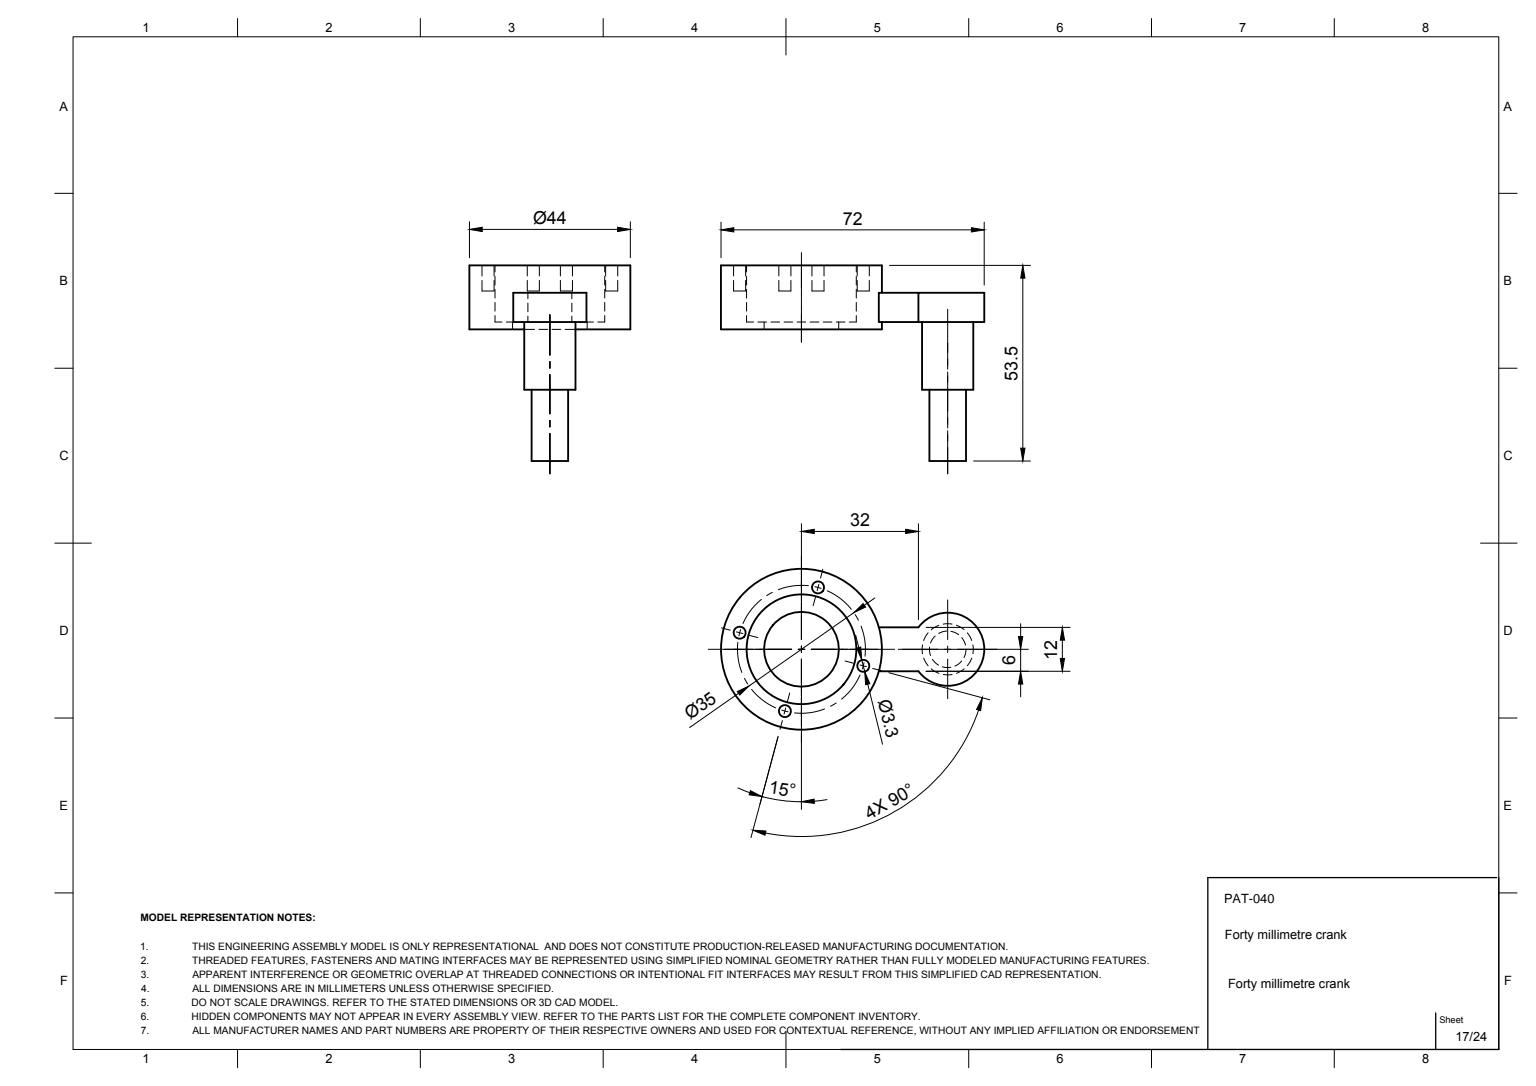
ISO-10303-21;
HEADER;
/* Generated by software containing ST-Developer
 * from STEP Tools, Inc. (www.steptools.com) 
 */

FILE_DESCRIPTION(
/* description */ ('Four-bar tabletop demonstrator'),
/* implementation_level */ '2;1');

FILE_NAME(
/* name */ 'Forty millimetre crank.step',
/* time_stamp */ '2026-10-29T17:05:23-07:00',
/* author */ (''),
/* organization */ (''),
/* preprocessor_version */ 'ST-DEVELOPER v20.2',
/* originating_system */ 'Autodesk Translation Framework v15.17.0.0',
/* authorisation */ '');

FILE_SCHEMA (('AUTOMOTIVE_DESIGN { 1 0 10303 214 3 1 1 }'));
ENDSEC;

DATA;
#10=MECHANICAL_DESIGN_GEOMETRIC_PRESENTATION_REPRESENTATION('',(#340),#6705);
#310=SHAPE_REPRESENTATION_RELATIONSHIP('SRR','None',#6818,#325);
#325=ADVANCED_BREP_SHAPE_REPRESENTATION('',(#362),#6691);
#340=STYLED_ITEM('',(#7003),#362);
#362=MANIFOLD_SOLID_BREP('Body1',#3385);
#416=FACE_BOUND('',#869,.T.);
#417=FACE_BOUND('',#872,.T.);
#418=FACE_BOUND('',#874,.T.);
#419=FACE_BOUND('',#875,.T.);
#420=FACE_BOUND('',#876,.T.);
#421=FACE_BOUND('',#877,.T.);
#422=FACE_BOUND('',#878,.T.);
#423=FACE_BOUND('',#880,.T.);
#424=FACE_BOUND('',#886,.T.);
#425=FACE_BOUND('',#888,.T.);
#491=PLANE('',#3705);
#492=PLANE('',#3709);
#493=PLANE('',#3713);
#494=PLANE('',#3717);
#495=PLANE('',#3721);
#496=PLANE('',#3730);
#497=PLANE('',#3731);
#498=PLANE('',#3732);
#499=PLANE('',#3733);
#500=PLANE('',#3735);
#501=PLANE('',#3738);
#502=PLANE('',#3740);
#503=PLANE('',#3746);
#621=FACE_OUTER_BOUND('',#859,.T.);
#622=FACE_OUTER_BOUND('',#860,.T.);
#623=FACE_OUTER_BOUND('',#861,.T.);
#624=FACE_OUTER_BOUND('',#862,.T.);
#625=FACE_OUTER_BOUND('',#863,.T.);
#626=FACE_OUTER_BOUND('',#864,.T.);
#627=FACE_OUTER_BOUND('',#865,.T.);
#628=FACE_OUTER_BOUND('',#866,.T.);
#629=FACE_OUTER_BOUND('',#867,.T.);
#630=FACE_OUTER_BOUND('',#868,.T.);
#631=FACE_OUTER_BOUND('',#870,.T.);
#632=FACE_OUTER_BOUND('',#871,.T.);
#633=FACE_OUTER_BOUND('',#873,.T.);
#634=FACE_OUTER_BOUND('',#879,.T.);
#635=FACE_OUTER_BOUND('',#881,.T.);
#636=FACE_OUTER_BOUND('',#882,.T.);
#637=FACE_OUTER_BOUND('',#883,.T.);
#638=FACE_OUTER_BOUND('',#884,.T.);
#639=FACE_OUTER_BOUND('',#885,.T.);
#640=FACE_OUTER_BOUND('',#887,.T.);
#641=FACE_OUTER_BOUND('',#889,.T.);
#642=FACE_OUTER_BOUND('',#890,.T.);
#643=FACE_OUTER_BOUND('',#891,.T.);
#859=EDGE_LOOP('',(#2550,#2551,#2552,#2553));
#860=EDGE_LOOP('',(#2554));
#861=EDGE_LOOP('',(#2555,#2556,#2557,#2558));
#862=EDGE_LOOP('',(#2559));
#863=EDGE_LOOP('',(#2560,#2561,#2562,#2563));
#864=EDGE_LOOP('',(#2564));
#865=EDGE_LOOP('',(#2565,#2566,#2567,#2568));
#866=EDGE_LOOP('',(#2569));
#867=EDGE_LOOP('',(#2570,#2571,#2572,#2573));
#868=EDGE_LOOP('',(#2574));
#869=EDGE_LOOP('',(#2575));
#870=EDGE_LOOP('',(#2576,#2577,#2578,#2579));
#871=EDGE_LOOP('',(#2580,#2581,#2582,#2583));
#872=EDGE_LOOP('',(#2584,#2585,#2586,#2587));
#873=EDGE_LOOP('',(#2588));
#874=EDGE_LOOP('',(#2589));
#875=EDGE_LOOP('',(#2590));
#876=EDGE_LOOP('',(#2591));
#877=EDGE_LOOP('',(#2592));
#878=EDGE_LOOP('',(#2593));
#879=EDGE_LOOP('',(#2594));
#880=EDGE_LOOP('',(#2595));
#881=EDGE_LOOP('',(#2596,#2597,#2598,#2599));
#882=EDGE_LOOP('',(#2600,#2601,#2602,#2603));
#883=EDGE_LOOP('',(#2604,#2605,#2606,#2607));
#884=EDGE_LOOP('',(#2608,#2609,#2610,#2611));
#885=EDGE_LOOP('',(#2612,#2613,#2614,#2615));
#886=EDGE_LOOP('',(#2616));
#887=EDGE_LOOP('',(#2617));
#888=EDGE_LOOP('',(#2618));
#889=EDGE_LOOP('',(#2619,#2620,#2621,#2622));
#890=EDGE_LOOP('',(#2623,#2624,#2625,#2626));
#891=EDGE_LOOP('',(#2627));
#1113=LINE('',#5581,#1283);
#1114=LINE('',#5588,#1284);
#1115=LINE('',#5595,#1285);
#1116=LINE('',#5602,#1286);
#1117=LINE('',#5609,#1287);
#1118=LINE('',#5617,#1288);
#1119=LINE('',#5622,#1289);
#1120=LINE('',#5626,#1290);
#1121=LINE('',#5630,#1291);
#1122=LINE('',#5636,#1292);
#1123=LINE('',#5638,#1293);
#1124=LINE('',#5639,#1294);
#1125=LINE('',#5642,#1295);
#1126=LINE('',#5646,#1296);
#1127=LINE('',#5647,#1297);
#1128=LINE('',#5659,#1298);
#1129=LINE('',#5662,#1299);
#1283=VECTOR('',#4394,0.165);
#1284=VECTOR('',#4403,0.165);
#1285=VECTOR('',#4412,0.165);
#1286=VECTOR('',#4421,0.165);
#1287=VECTOR('',#4430,1.5);
#1288=VECTOR('',#4441,1.02);
#1289=VECTOR('',#4446,2.2);
#1290=VECTOR('',#4449,1.);
#1291=VECTOR('',#4452,1.);
#1292=VECTOR('',#4461,1.);
#1293=VECTOR('',#4462,1.);
#1294=VECTOR('',#4463,1.);
#1295=VECTOR('',#4466,1.);
#1296=VECTOR('',#4471,1.);
#1297=VECTOR('',#4472,1.);
#1298=VECTOR('',#4489,0.7);
#1299=VECTOR('',#4492,0.5);
#1452=CIRCLE('',#3703,0.165);
#1453=CIRCLE('',#3704,0.165);
#1454=CIRCLE('',#3707,0.165);
#1455=CIRCLE('',#3708,0.165);
#1456=CIRCLE('',#3711,0.165);
#1457=CIRCLE('',#3712,0.165);
#1458=CIRCLE('',#3715,0.165);
#1459=CIRCLE('',#3716,0.165);
#1460=CIRCLE('',#3719,1.5);
#1461=CIRCLE('',#3720,1.5);
#1462=CIRCLE('',#3722,1.02);
#1463=CIRCLE('',#3724,1.02);
#1464=CIRCLE('',#3726,2.2);
#1465=CIRCLE('',#3727,2.2);
#1466=CIRCLE('',#3728,2.2);
#1467=CIRCLE('',#3729,2.2);
#1468=CIRCLE('',#3734,1.);
#1469=CIRCLE('',#3737,1.);
#1470=CIRCLE('',#3739,0.7);
#1471=CIRCLE('',#3741,0.7);
#1472=CIRCLE('',#3742,0.5);
#1473=CIRCLE('',#3745,0.5);
#1687=VERTEX_POINT('',#5578);
#1688=VERTEX_POINT('',#5580);
#1689=VERTEX_POINT('',#5585);
#1690=VERTEX_POINT('',#5587);
#1691=VERTEX_POINT('',#5592);
#1692=VERTEX_POINT('',#5594);
#1693=VERTEX_POINT('',#5599);
#1694=VERTEX_POINT('',#5601);
#1695=VERTEX_POINT('',#5606);
#1696=VERTEX_POINT('',#5608);
#1697=VERTEX_POINT('',#5612);
#1698=VERTEX_POINT('',#5615);
#1699=VERTEX_POINT('',#5619);
#1700=VERTEX_POINT('',#5621);
#1701=VERTEX_POINT('',#5624);
#1702=VERTEX_POINT('',#5625);
#1703=VERTEX_POINT('',#5627);
#1704=VERTEX_POINT('',#5629);
#1705=VERTEX_POINT('',#5635);
#1706=VERTEX_POINT('',#5637);
#1707=VERTEX_POINT('',#5641);
#1708=VERTEX_POINT('',#5645);
#1709=VERTEX_POINT('',#5651);
#1710=VERTEX_POINT('',#5654);
#1711=VERTEX_POINT('',#5656);
#1712=VERTEX_POINT('',#5661);
#2011=EDGE_CURVE('',#1687,#1687,#1452,.T.);
#2012=EDGE_CURVE('',#1687,#1688,#1113,.T.);
#2013=EDGE_CURVE('',#1688,#1688,#1453,.T.);
#2014=EDGE_CURVE('',#1689,#1689,#1454,.T.);
#2015=EDGE_CURVE('',#1689,#1690,#1114,.T.);
#2016=EDGE_CURVE('',#1690,#1690,#1455,.T.);
#2017=EDGE_CURVE('',#1691,#1691,#1456,.T.);
#2018=EDGE_CURVE('',#1691,#1692,#1115,.T.);
#2019=EDGE_CURVE('',#1692,#1692,#1457,.T.);
#2020=EDGE_CURVE('',#1693,#1693,#1458,.T.);
#2021=EDGE_CURVE('',#1693,#1694,#1116,.T.);
#2022=EDGE_CURVE('',#1694,#1694,#1459,.T.);
#2023=EDGE_CURVE('',#1695,#1695,#1460,.T.);
#2024=EDGE_CURVE('',#1695,#1696,#1117,.T.);
#2025=EDGE_CURVE('',#1696,#1696,#1461,.T.);
#2026=EDGE_CURVE('',#1697,#1697,#1462,.T.);
#2027=EDGE_CURVE('',#1698,#1698,#1463,.T.);
#2028=EDGE_CURVE('',#1698,#1697,#1118,.T.);
#2029=EDGE_CURVE('',#1699,#1699,#1464,.T.);
#2030=EDGE_CURVE('',#1699,#1700,#1119,.T.);
#2031=EDGE_CURVE('',#1700,#1700,#1465,.T.);
#2032=EDGE_CURVE('',#1701,#1702,#1120,.T.);
#2033=EDGE_CURVE('',#1703,#1701,#1466,.T.);
#2034=EDGE_CURVE('',#1704,#1703,#1121,.T.);
#2035=EDGE_CURVE('',#1702,#1704,#1467,.T.);
#2036=EDGE_CURVE('',#1705,#1703,#1122,.T.);
#2037=EDGE_CURVE('',#1706,#1705,#1123,.T.);
#2038=EDGE_CURVE('',#1704,#1706,#1124,.T.);
#2039=EDGE_CURVE('',#1701,#1707,#1125,.T.);
#2040=EDGE_CURVE('',#1707,#1705,#1468,.T.);
#2041=EDGE_CURVE('',#1708,#1702,#1126,.T.);
#2042=EDGE_CURVE('',#1707,#1708,#1127,.T.);
#2043=EDGE_CURVE('',#1708,#1706,#1469,.T.);
#2044=EDGE_CURVE('',#1709,#1709,#1470,.T.);
#2045=EDGE_CURVE('',#1710,#1710,#1471,.T.);
#2046=EDGE_CURVE('',#1711,#1711,#1472,.T.);
#2047=EDGE_CURVE('',#1709,#1710,#1128,.T.);
#2048=EDGE_CURVE('',#1711,#1712,#1129,.T.);
#2049=EDGE_CURVE('',#1712,#1712,#1473,.T.);
#2550=ORIENTED_EDGE('',*,*,#2011,.F.);
#2551=ORIENTED_EDGE('',*,*,#2012,.T.);
#2552=ORIENTED_EDGE('',*,*,#2013,.F.);
#2553=ORIENTED_EDGE('',*,*,#2012,.F.);
#2554=ORIENTED_EDGE('',*,*,#2011,.T.);
#2555=ORIENTED_EDGE('',*,*,#2014,.F.);
#2556=ORIENTED_EDGE('',*,*,#2015,.T.);
#2557=ORIENTED_EDGE('',*,*,#2016,.F.);
#2558=ORIENTED_EDGE('',*,*,#2015,.F.);
#2559=ORIENTED_EDGE('',*,*,#2014,.T.);
#2560=ORIENTED_EDGE('',*,*,#2017,.F.);
#2561=ORIENTED_EDGE('',*,*,#2018,.T.);
#2562=ORIENTED_EDGE('',*,*,#2019,.F.);
#2563=ORIENTED_EDGE('',*,*,#2018,.F.);
#2564=ORIENTED_EDGE('',*,*,#2017,.T.);
#2565=ORIENTED_EDGE('',*,*,#2020,.F.);
#2566=ORIENTED_EDGE('',*,*,#2021,.T.);
#2567=ORIENTED_EDGE('',*,*,#2022,.F.);
#2568=ORIENTED_EDGE('',*,*,#2021,.F.);
#2569=ORIENTED_EDGE('',*,*,#2020,.T.);
#2570=ORIENTED_EDGE('',*,*,#2023,.F.);
#2571=ORIENTED_EDGE('',*,*,#2024,.T.);
#2572=ORIENTED_EDGE('',*,*,#2025,.F.);
#2573=ORIENTED_EDGE('',*,*,#2024,.F.);
#2574=ORIENTED_EDGE('',*,*,#2023,.T.);
#2575=ORIENTED_EDGE('',*,*,#2026,.F.);
#2576=ORIENTED_EDGE('',*,*,#2027,.F.);
#2577=ORIENTED_EDGE('',*,*,#2028,.T.);
#2578=ORIENTED_EDGE('',*,*,#2026,.T.);
#2579=ORIENTED_EDGE('',*,*,#2028,.F.);
#2580=ORIENTED_EDGE('',*,*,#2029,.F.);
#2581=ORIENTED_EDGE('',*,*,#2030,.T.);
#2582=ORIENTED_EDGE('',*,*,#2031,.T.);
#2583=ORIENTED_EDGE('',*,*,#2030,.F.);
#2584=ORIENTED_EDGE('',*,*,#2032,.F.);
#2585=ORIENTED_EDGE('',*,*,#2033,.F.);
#2586=ORIENTED_EDGE('',*,*,#2034,.F.);
#2587=ORIENTED_EDGE('',*,*,#2035,.F.);
#2588=ORIENTED_EDGE('',*,*,#2029,.T.);
#2589=ORIENTED_EDGE('',*,*,#2025,.T.);
#2590=ORIENTED_EDGE('',*,*,#2022,.T.);
#2591=ORIENTED_EDGE('',*,*,#2019,.T.);
#2592=ORIENTED_EDGE('',*,*,#2016,.T.);
#2593=ORIENTED_EDGE('',*,*,#2013,.T.);
#2594=ORIENTED_EDGE('',*,*,#2031,.F.);
#2595=ORIENTED_EDGE('',*,*,#2027,.T.);
#2596=ORIENTED_EDGE('',*,*,#2034,.T.);
#2597=ORIENTED_EDGE('',*,*,#2036,.F.);
#2598=ORIENTED_EDGE('',*,*,#2037,.F.);
#2599=ORIENTED_EDGE('',*,*,#2038,.F.);
#2600=ORIENTED_EDGE('',*,*,#2033,.T.);
#2601=ORIENTED_EDGE('',*,*,#2039,.T.);
#2602=ORIENTED_EDGE('',*,*,#2040,.T.);
#2603=ORIENTED_EDGE('',*,*,#2036,.T.);
#2604=ORIENTED_EDGE('',*,*,#2032,.T.);
#2605=ORIENTED_EDGE('',*,*,#2041,.F.);
#2606=ORIENTED_EDGE('',*,*,#2042,.F.);
#2607=ORIENTED_EDGE('',*,*,#2039,.F.);
#2608=ORIENTED_EDGE('',*,*,#2042,.T.);
#2609=ORIENTED_EDGE('',*,*,#2043,.T.);
#2610=ORIENTED_EDGE('',*,*,#2037,.T.);
#2611=ORIENTED_EDGE('',*,*,#2040,.F.);
#2612=ORIENTED_EDGE('',*,*,#2035,.T.);
#2613=ORIENTED_EDGE('',*,*,#2038,.T.);
#2614=ORIENTED_EDGE('',*,*,#2043,.F.);
#2615=ORIENTED_EDGE('',*,*,#2041,.T.);
#2616=ORIENTED_EDGE('',*,*,#2044,.T.);
#2617=ORIENTED_EDGE('',*,*,#2045,.F.);
#2618=ORIENTED_EDGE('',*,*,#2046,.F.);
#2619=ORIENTED_EDGE('',*,*,#2044,.F.);
#2620=ORIENTED_EDGE('',*,*,#2047,.T.);
#2621=ORIENTED_EDGE('',*,*,#2045,.T.);
#2622=ORIENTED_EDGE('',*,*,#2047,.F.);
#2623=ORIENTED_EDGE('',*,*,#2046,.T.);
#2624=ORIENTED_EDGE('',*,*,#2048,.T.);
#2625=ORIENTED_EDGE('',*,*,#2049,.T.);
#2626=ORIENTED_EDGE('',*,*,#2048,.F.);
#2627=ORIENTED_EDGE('',*,*,#2049,.F.);
#3131=CYLINDRICAL_SURFACE('',#3702,0.165);
#3132=CYLINDRICAL_SURFACE('',#3706,0.165);
#3133=CYLINDRICAL_SURFACE('',#3710,0.165);
#3134=CYLINDRICAL_SURFACE('',#3714,0.165);
#3135=CYLINDRICAL_SURFACE('',#3718,1.5);
#3136=CYLINDRICAL_SURFACE('',#3723,1.02);
#3137=CYLINDRICAL_SURFACE('',#3725,2.2);
#3138=CYLINDRICAL_SURFACE('',#3736,1.);
#3139=CYLINDRICAL_SURFACE('',#3743,0.7);
#3140=CYLINDRICAL_SURFACE('',#3744,0.5);
#3237=ADVANCED_FACE('',(#621),#3131,.F.);
#3238=ADVANCED_FACE('',(#622),#491,.T.);
#3239=ADVANCED_FACE('',(#623),#3132,.F.);
#3240=ADVANCED_FACE('',(#624),#492,.T.);
#3241=ADVANCED_FACE('',(#625),#3133,.F.);
#3242=ADVANCED_FACE('',(#626),#493,.T.);
#3243=ADVANCED_FACE('',(#627),#3134,.F.);
#3244=ADVANCED_FACE('',(#628),#494,.T.);
#3245=ADVANCED_FACE('',(#629),#3135,.F.);
#3246=ADVANCED_FACE('',(#630,#416),#495,.T.);
#3247=ADVANCED_FACE('',(#631),#3136,.F.);
#3248=ADVANCED_FACE('',(#632,#417),#3137,.T.);
#3249=ADVANCED_FACE('',(#633,#418,#419,#420,#421,#422),#496,.T.);
#3250=ADVANCED_FACE('',(#634,#423),#497,.F.);
#3251=ADVANCED_FACE('',(#635),#498,.T.);
#3252=ADVANCED_FACE('',(#636),#499,.T.);
#3253=ADVANCED_FACE('',(#637),#500,.T.);
#3254=ADVANCED_FACE('',(#638),#3138,.T.);
#3255=ADVANCED_FACE('',(#639,#424),#501,.F.);
#3256=ADVANCED_FACE('',(#640,#425),#502,.F.);
#3257=ADVANCED_FACE('',(#641),#3139,.T.);
#3258=ADVANCED_FACE('',(#642),#3140,.T.);
#3259=ADVANCED_FACE('',(#643),#503,.F.);
#3385=CLOSED_SHELL('',(#3237,#3238,#3239,#3240,#3241,#3242,#3243,#3244,
#3245,#3246,#3247,#3248,#3249,#3250,#3251,#3252,#3253,#3254,#3255,#3256,
#3257,#3258,#3259));
#3701=AXIS2_PLACEMENT_3D('',#5576,#4388,#4389);
#3702=AXIS2_PLACEMENT_3D('',#5577,#4390,#4391);
#3703=AXIS2_PLACEMENT_3D('',#5579,#4392,#4393);
#3704=AXIS2_PLACEMENT_3D('',#5582,#4395,#4396);
#3705=AXIS2_PLACEMENT_3D('',#5583,#4397,#4398);
#3706=AXIS2_PLACEMENT_3D('',#5584,#4399,#4400);
#3707=AXIS2_PLACEMENT_3D('',#5586,#4401,#4402);
#3708=AXIS2_PLACEMENT_3D('',#5589,#4404,#4405);
#3709=AXIS2_PLACEMENT_3D('',#5590,#4406,#4407);
#3710=AXIS2_PLACEMENT_3D('',#5591,#4408,#4409);
#3711=AXIS2_PLACEMENT_3D('',#5593,#4410,#4411);
#3712=AXIS2_PLACEMENT_3D('',#5596,#4413,#4414);
#3713=AXIS2_PLACEMENT_3D('',#5597,#4415,#4416);
#3714=AXIS2_PLACEMENT_3D('',#5598,#4417,#4418);
#3715=AXIS2_PLACEMENT_3D('',#5600,#4419,#4420);
#3716=AXIS2_PLACEMENT_3D('',#5603,#4422,#4423);
#3717=AXIS2_PLACEMENT_3D('',#5604,#4424,#4425);
#3718=AXIS2_PLACEMENT_3D('',#5605,#4426,#4427);
#3719=AXIS2_PLACEMENT_3D('',#5607,#4428,#4429);
#3720=AXIS2_PLACEMENT_3D('',#5610,#4431,#4432);
#3721=AXIS2_PLACEMENT_3D('',#5611,#4433,#4434);
#3722=AXIS2_PLACEMENT_3D('',#5613,#4435,#4436);
#3723=AXIS2_PLACEMENT_3D('',#5614,#4437,#4438);
#3724=AXIS2_PLACEMENT_3D('',#5616,#4439,#4440);
#3725=AXIS2_PLACEMENT_3D('',#5618,#4442,#4443);
#3726=AXIS2_PLACEMENT_3D('',#5620,#4444,#4445);
#3727=AXIS2_PLACEMENT_3D('',#5623,#4447,#4448);
#3728=AXIS2_PLACEMENT_3D('',#5628,#4450,#4451);
#3729=AXIS2_PLACEMENT_3D('',#5631,#4453,#4454);
#3730=AXIS2_PLACEMENT_3D('',#5632,#4455,#4456);
#3731=AXIS2_PLACEMENT_3D('',#5633,#4457,#4458);
#3732=AXIS2_PLACEMENT_3D('',#5634,#4459,#4460);
#3733=AXIS2_PLACEMENT_3D('',#5640,#4464,#4465);
#3734=AXIS2_PLACEMENT_3D('',#5643,#4467,#4468);
#3735=AXIS2_PLACEMENT_3D('',#5644,#4469,#4470);
#3736=AXIS2_PLACEMENT_3D('',#5648,#4473,#4474);
#3737=AXIS2_PLACEMENT_3D('',#5649,#4475,#4476);
#3738=AXIS2_PLACEMENT_3D('',#5650,#4477,#4478);
#3739=AXIS2_PLACEMENT_3D('',#5652,#4479,#4480);
#3740=AXIS2_PLACEMENT_3D('',#5653,#4481,#4482);
#3741=AXIS2_PLACEMENT_3D('',#5655,#4483,#4484);
#3742=AXIS2_PLACEMENT_3D('',#5657,#4485,#4486);
#3743=AXIS2_PLACEMENT_3D('',#5658,#4487,#4488);
#3744=AXIS2_PLACEMENT_3D('',#5660,#4490,#4491);
#3745=AXIS2_PLACEMENT_3D('',#5663,#4493,#4494);
#3746=AXIS2_PLACEMENT_3D('',#5664,#4495,#4496);
#4388=DIRECTION('axis',(0.,0.,1.));
#4389=DIRECTION('refdir',(1.,0.,0.));
#4390=DIRECTION('center_axis',(0.,0.,1.));
#4391=DIRECTION('ref_axis',(1.,0.,0.));
#4392=DIRECTION('center_axis',(0.,0.,1.));
#4393=DIRECTION('ref_axis',(1.,0.,0.));
#4394=DIRECTION('',(0.,0.,1.));
#4395=DIRECTION('center_axis',(0.,0.,-1.));
#4396=DIRECTION('ref_axis',(1.,0.,0.));
#4397=DIRECTION('center_axis',(0.,0.,1.));
#4398=DIRECTION('ref_axis',(1.,0.,0.));
#4399=DIRECTION('center_axis',(0.,0.,1.));
#4400=DIRECTION('ref_axis',(1.,0.,0.));
#4401=DIRECTION('center_axis',(0.,0.,1.));
#4402=DIRECTION('ref_axis',(1.,0.,0.));
#4403=DIRECTION('',(0.,0.,1.));
#4404=DIRECTION('center_axis',(0.,0.,-1.));
#4405=DIRECTION('ref_axis',(1.,0.,0.));
#4406=DIRECTION('center_axis',(0.,0.,1.));
#4407=DIRECTION('ref_axis',(1.,0.,0.));
#4408=DIRECTION('center_axis',(0.,0.,1.));
#4409=DIRECTION('ref_axis',(1.,0.,0.));
#4410=DIRECTION('center_axis',(0.,0.,1.));
#4411=DIRECTION('ref_axis',(1.,0.,0.));
#4412=DIRECTION('',(0.,0.,1.));
#4413=DIRECTION('center_axis',(0.,0.,-1.));
#4414=DIRECTION('ref_axis',(1.,0.,0.));
#4415=DIRECTION('center_axis',(0.,0.,1.));
#4416=DIRECTION('ref_axis',(1.,0.,0.));
#4417=DIRECTION('center_axis',(0.,0.,1.));
#4418=DIRECTION('ref_axis',(1.,0.,0.));
#4419=DIRECTION('center_axis',(0.,0.,1.));
#4420=DIRECTION('ref_axis',(1.,0.,0.));
#4421=DIRECTION('',(0.,0.,1.));
#4422=DIRECTION('center_axis',(0.,0.,-1.));
#4423=DIRECTION('ref_axis',(1.,0.,0.));
#4424=DIRECTION('center_axis',(0.,0.,1.));
#4425=DIRECTION('ref_axis',(1.,0.,0.));
#4426=DIRECTION('center_axis',(0.,0.,1.));
#4427=DIRECTION('ref_axis',(1.,0.,0.));
#4428=DIRECTION('center_axis',(0.,0.,1.));
#4429=DIRECTION('ref_axis',(1.,0.,0.));
#4430=DIRECTION('',(0.,0.,1.));
#4431=DIRECTION('center_axis',(0.,0.,-1.));
#4432=DIRECTION('ref_axis',(1.,0.,0.));
#4433=DIRECTION('center_axis',(0.,0.,1.));
#4434=DIRECTION('ref_axis',(1.,0.,0.));
#4435=DIRECTION('center_axis',(0.,0.,1.));
#4436=DIRECTION('ref_axis',(1.,0.,0.));
#4437=DIRECTION('center_axis',(0.,0.,1.));
#4438=DIRECTION('ref_axis',(1.,0.,0.));
#4439=DIRECTION('center_axis',(0.,0.,1.));
#4440=DIRECTION('ref_axis',(1.,0.,0.));
#4441=DIRECTION('',(0.,0.,1.));
#4442=DIRECTION('center_axis',(0.,0.,1.));
#4443=DIRECTION('ref_axis',(1.,0.,0.));
#4444=DIRECTION('center_axis',(0.,0.,1.));
#4445=DIRECTION('ref_axis',(1.,0.,0.));
#4446=DIRECTION('',(0.,0.,-1.));
#4447=DIRECTION('center_axis',(0.,0.,1.));
#4448=DIRECTION('ref_axis',(1.,0.,0.));
#4449=DIRECTION('',(0.,0.,-1.));
#4450=DIRECTION('center_axis',(0.,0.,-1.));
#4451=DIRECTION('ref_axis',(1.,0.,0.));
#4452=DIRECTION('',(0.,0.,1.));
#4453=DIRECTION('center_axis',(0.,0.,1.));
#4454=DIRECTION('ref_axis',(1.,0.,0.));
#4455=DIRECTION('center_axis',(0.,0.,1.));
#4456=DIRECTION('ref_axis',(1.,0.,0.));
#4457=DIRECTION('center_axis',(0.,0.,1.));
#4458=DIRECTION('ref_axis',(1.,0.,0.));
#4459=DIRECTION('center_axis',(0.866025403784439,-0.5,0.));
#4460=DIRECTION('ref_axis',(0.5,0.866025403784439,0.));
#4461=DIRECTION('',(0.5,0.866025403784439,0.));
#4462=DIRECTION('',(0.,0.,1.));
#4463=DIRECTION('',(-0.5,-0.866025403784439,0.));
#4464=DIRECTION('center_axis',(0.,0.,1.));
#4465=DIRECTION('ref_axis',(1.,0.,0.));
#4466=DIRECTION('',(-0.5,-0.866025403784439,0.));
#4467=DIRECTION('center_axis',(0.,0.,1.));
#4468=DIRECTION('ref_axis',(1.,0.,0.));
#4469=DIRECTION('center_axis',(-0.866025403784439,0.5,0.));
#4470=DIRECTION('ref_axis',(-0.5,-0.866025403784439,0.));
#4471=DIRECTION('',(0.5,0.866025403784439,0.));
#4472=DIRECTION('',(0.,0.,-1.));
#4473=DIRECTION('center_axis',(0.,0.,1.));
#4474=DIRECTION('ref_axis',(-0.5,-0.866025403784438,0.));
#4475=DIRECTION('center_axis',(0.,0.,1.));
#4476=DIRECTION('ref_axis',(1.,0.,0.));
#4477=DIRECTION('center_axis',(0.,0.,1.));
#4478=DIRECTION('ref_axis',(1.,0.,0.));
#4479=DIRECTION('center_axis',(0.,0.,1.));
#4480=DIRECTION('ref_axis',(1.,0.,0.));
#4481=DIRECTION('center_axis',(0.,0.,1.));
#4482=DIRECTION('ref_axis',(1.,0.,0.));
#4483=DIRECTION('center_axis',(0.,0.,1.));
#4484=DIRECTION('ref_axis',(1.,0.,0.));
#4485=DIRECTION('center_axis',(0.,0.,-1.));
#4486=DIRECTION('ref_axis',(1.,0.,0.));
#4487=DIRECTION('center_axis',(0.,0.,1.));
#4488=DIRECTION('ref_axis',(1.,0.,0.));
#4489=DIRECTION('',(0.,0.,-1.));
#4490=DIRECTION('center_axis',(0.,0.,1.));
#4491=DIRECTION('ref_axis',(1.,0.,0.));
#4492=DIRECTION('',(0.,0.,-1.));
#4493=DIRECTION('center_axis',(0.,0.,1.));
#4494=DIRECTION('ref_axis',(1.,0.,0.));
#4495=DIRECTION('center_axis',(0.,0.,1.));
#4496=DIRECTION('ref_axis',(1.,0.,0.));
#5576=CARTESIAN_POINT('',(0.,0.,0.));
#5577=CARTESIAN_POINT('Origin',(0.762563132923542,2.2266647480613,5.65));
#5578=CARTESIAN_POINT('',(0.597563132923542,2.2266647480613,5.65));
#5579=CARTESIAN_POINT('Origin',(0.762563132923542,2.2266647480613,5.65));
#5580=CARTESIAN_POINT('',(0.597563132923542,2.2266647480613,6.35));
#5581=CARTESIAN_POINT('',(0.597563132923542,2.2266647480613,5.65));
#5582=CARTESIAN_POINT('Origin',(0.762563132923542,2.2266647480613,6.35));
#5583=CARTESIAN_POINT('Origin',(0.762563132923542,2.2266647480613,5.65));
#5584=CARTESIAN_POINT('Origin',(0.762563132923542,4.70153848221421,5.65));
#5585=CARTESIAN_POINT('',(0.597563132923542,4.70153848221421,5.65));
#5586=CARTESIAN_POINT('Origin',(0.762563132923542,4.70153848221421,5.65));
#5587=CARTESIAN_POINT('',(0.597563132923542,4.70153848221421,6.35));
#5588=CARTESIAN_POINT('',(0.597563132923542,4.70153848221421,5.65));
#5589=CARTESIAN_POINT('Origin',(0.762563132923542,4.70153848221421,6.35));
#5590=CARTESIAN_POINT('Origin',(0.762563132923542,4.70153848221421,5.65));
#5591=CARTESIAN_POINT('Origin',(3.23743686707646,4.70153848221421,5.65));
#5592=CARTESIAN_POINT('',(3.07243686707646,4.70153848221421,5.65));
#5593=CARTESIAN_POINT('Origin',(3.23743686707646,4.70153848221421,5.65));
#5594=CARTESIAN_POINT('',(3.07243686707646,4.70153848221421,6.35));
#5595=CARTESIAN_POINT('',(3.07243686707646,4.70153848221421,5.65));
#5596=CARTESIAN_POINT('Origin',(3.23743686707646,4.70153848221421,6.35));
#5597=CARTESIAN_POINT('Origin',(3.23743686707646,4.70153848221421,5.65));
#5598=CARTESIAN_POINT('Origin',(3.23743686707646,2.2266647480613,5.65));
#5599=CARTESIAN_POINT('',(3.07243686707646,2.2266647480613,5.65));
#5600=CARTESIAN_POINT('Origin',(3.23743686707646,2.2266647480613,5.65));
#5601=CARTESIAN_POINT('',(3.07243686707646,2.2266647480613,6.35));
#5602=CARTESIAN_POINT('',(3.07243686707646,2.2266647480613,5.65));
#5603=CARTESIAN_POINT('Origin',(3.23743686707646,2.2266647480613,6.35));
#5604=CARTESIAN_POINT('Origin',(3.23743686707646,2.2266647480613,5.65));
#5605=CARTESIAN_POINT('Origin',(2.,3.46410161513775,4.8));
#5606=CARTESIAN_POINT('',(0.5,3.46410161513775,4.8));
#5607=CARTESIAN_POINT('Origin',(2.,3.46410161513775,4.8));
#5608=CARTESIAN_POINT('',(0.5,3.46410161513775,6.35));
#5609=CARTESIAN_POINT('',(0.5,3.46410161513775,4.8));
#5610=CARTESIAN_POINT('Origin',(2.,3.46410161513775,6.35));
#5611=CARTESIAN_POINT('Origin',(2.,3.46410161513775,4.8));
#5612=CARTESIAN_POINT('',(0.98,3.46410161513775,4.8));
#5613=CARTESIAN_POINT('Origin',(2.,3.46410161513775,4.8));
#5614=CARTESIAN_POINT('Origin',(2.,3.46410161513775,4.5));
#5615=CARTESIAN_POINT('',(0.98,3.46410161513775,4.6));
#5616=CARTESIAN_POINT('Origin',(2.,3.46410161513775,4.6));
#5617=CARTESIAN_POINT('',(0.98,3.46410161513775,4.5));
#5618=CARTESIAN_POINT('Origin',(2.,3.46410161513775,4.6));
#5619=CARTESIAN_POINT('',(-0.2,3.46410161513775,6.35));
#5620=CARTESIAN_POINT('Origin',(2.,3.46410161513775,6.35));
#5621=CARTESIAN_POINT('',(-0.2,3.46410161513775,4.6));
#5622=CARTESIAN_POINT('',(-0.2,3.46410161513775,4.6));
#5623=CARTESIAN_POINT('Origin',(2.,3.46410161513775,4.6));
#5624=CARTESIAN_POINT('',(0.422084233303501,1.93107133715542,5.6));
#5625=CARTESIAN_POINT('',(0.422084233303501,1.93107133715542,4.8));
#5626=CARTESIAN_POINT('',(0.4220842333035,1.93107133715542,4.6));
#5627=CARTESIAN_POINT('',(1.46131471784483,1.33107133715542,5.6));
#5628=CARTESIAN_POINT('Origin',(2.,3.46410161513775,5.6));
#5629=CARTESIAN_POINT('',(1.46131471784483,1.33107133715542,4.8));
#5630=CARTESIAN_POINT('',(1.46131471784483,1.33107133715542,4.6));
#5631=CARTESIAN_POINT('Origin',(2.,3.46410161513775,4.8));
#5632=CARTESIAN_POINT('Origin',(2.,3.46410161513775,6.35));
#5633=CARTESIAN_POINT('Origin',(2.,3.46410161513775,4.6));
#5634=CARTESIAN_POINT('Origin',(0.519615242270663,-0.3,4.8));
#5635=CARTESIAN_POINT('',(0.919615242270663,0.392820323027551,5.6));
#5636=CARTESIAN_POINT('',(2.51961524227066,3.16410161513775,5.6));
#5637=CARTESIAN_POINT('',(0.919615242270663,0.392820323027551,4.8));
#5638=CARTESIAN_POINT('',(0.919615242270663,0.392820323027551,4.8));
#5639=CARTESIAN_POINT('',(2.51961524227066,3.16410161513775,4.8));
#5640=CARTESIAN_POINT('Origin',(0.,0.,5.6));
#5641=CARTESIAN_POINT('',(-0.119615242270663,0.992820323027551,5.6));
#5642=CARTESIAN_POINT('',(-0.519615242270663,0.3,5.6));
#5643=CARTESIAN_POINT('Origin',(0.,0.,5.6));
#5644=CARTESIAN_POINT('Origin',(1.48038475772934,3.76410161513775,4.8));
#5645=CARTESIAN_POINT('',(-0.119615242270663,0.992820323027551,4.8));
#5646=CARTESIAN_POINT('',(-0.519615242270663,0.3,4.8));
#5647=CARTESIAN_POINT('',(-0.119615242270663,0.992820323027551,4.8));
#5648=CARTESIAN_POINT('Origin',(0.,0.,4.8));
#5649=CARTESIAN_POINT('Origin',(0.,0.,4.8));
#5650=CARTESIAN_POINT('Origin',(0.,0.,4.8));
#5651=CARTESIAN_POINT('',(-0.7,-8.57252759403147E-17,4.8));
#5652=CARTESIAN_POINT('Origin',(0.,0.,4.8));
#5653=CARTESIAN_POINT('Origin',(0.,0.,2.95));
#5654=CARTESIAN_POINT('',(-0.7,-8.57252759403147E-17,2.95));
#5655=CARTESIAN_POINT('Origin',(0.,0.,2.95));
#5656=CARTESIAN_POINT('',(-0.5,6.12323399573677E-17,2.95));
#5657=CARTESIAN_POINT('Origin',(0.,0.,2.95));
#5658=CARTESIAN_POINT('Origin',(0.,0.,2.95));
#5659=CARTESIAN_POINT('',(-0.7,-8.57252759403147E-17,2.95));
#5660=CARTESIAN_POINT('Origin',(0.,0.,1.));
#5661=CARTESIAN_POINT('',(-0.5,-6.12323399573677E-17,1.));
#5662=CARTESIAN_POINT('',(-0.5,-6.12323399573677E-17,1.));
#5663=CARTESIAN_POINT('Origin',(0.,0.,1.));
#5664=CARTESIAN_POINT('Origin',(0.,0.,1.));
#6669=UNCERTAINTY_MEASURE_WITH_UNIT(LENGTH_MEASURE(0.001),#6706,
'DISTANCE_ACCURACY_VALUE',
'Maximum model space distance between geometric entities at asserted c
onnectivities');
#6683=UNCERTAINTY_MEASURE_WITH_UNIT(LENGTH_MEASURE(0.001),#6706,
'DISTANCE_ACCURACY_VALUE',
'Maximum model space distance between geometric entities at asserted c
onnectivities');
#6691=(
GEOMETRIC_REPRESENTATION_CONTEXT(3)
GLOBAL_UNCERTAINTY_ASSIGNED_CONTEXT((#6669))
GLOBAL_UNIT_ASSIGNED_CONTEXT((#6706,#6708,#6709))
REPRESENTATION_CONTEXT('','3D')
);
#6705=(
GEOMETRIC_REPRESENTATION_CONTEXT(3)
GLOBAL_UNCERTAINTY_ASSIGNED_CONTEXT((#6683))
GLOBAL_UNIT_ASSIGNED_CONTEXT((#6706,#6708,#6709))
REPRESENTATION_CONTEXT('','3D')
);
#6706=(
LENGTH_UNIT()
NAMED_UNIT(*)
SI_UNIT(.CENTI.,.METRE.)
);
#6708=(
NAMED_UNIT(*)
PLANE_ANGLE_UNIT()
SI_UNIT($,.RADIAN.)
);
#6709=(
NAMED_UNIT(*)
SI_UNIT($,.STERADIAN.)
SOLID_ANGLE_UNIT()
);
#6717=SHAPE_DEFINITION_REPRESENTATION(#6738,#6818);
#6738=PRODUCT_DEFINITION_SHAPE('',$,#6840);
#6818=SHAPE_REPRESENTATION('',(#3701),#6691);
#6832=PRODUCT_DEFINITION_CONTEXT('part definition',#6897,'design');
#6840=PRODUCT_DEFINITION('Forty millimetre crank',
'Forty millimetre crank',#6861,#6832);
#6861=PRODUCT_DEFINITION_FORMATION('',$,#6906);
#6897=APPLICATION_CONTEXT(
'Core Data for Automotive Mechanical Design Process');
#6898=PRODUCT_CONTEXT('part definition',#6897,'mechanical');
#6906=PRODUCT('Forty millimetre crank','Forty millimetre crank',
'Forty millimetre crank',(#6898));
#6997=COLOUR_RGB('Off White',0.89,0.88,0.83);
#6998=FILL_AREA_STYLE_COLOUR('',#6997);
#6999=FILL_AREA_STYLE('',(#6998));
#7000=SURFACE_STYLE_FILL_AREA(#6999);
#7001=SURFACE_SIDE_STYLE('',(#7000));
#7002=SURFACE_STYLE_USAGE(.BOTH.,#7001);
#7003=PRESENTATION_STYLE_ASSIGNMENT((#7002));
ENDSEC;
END-ISO-10303-21;
